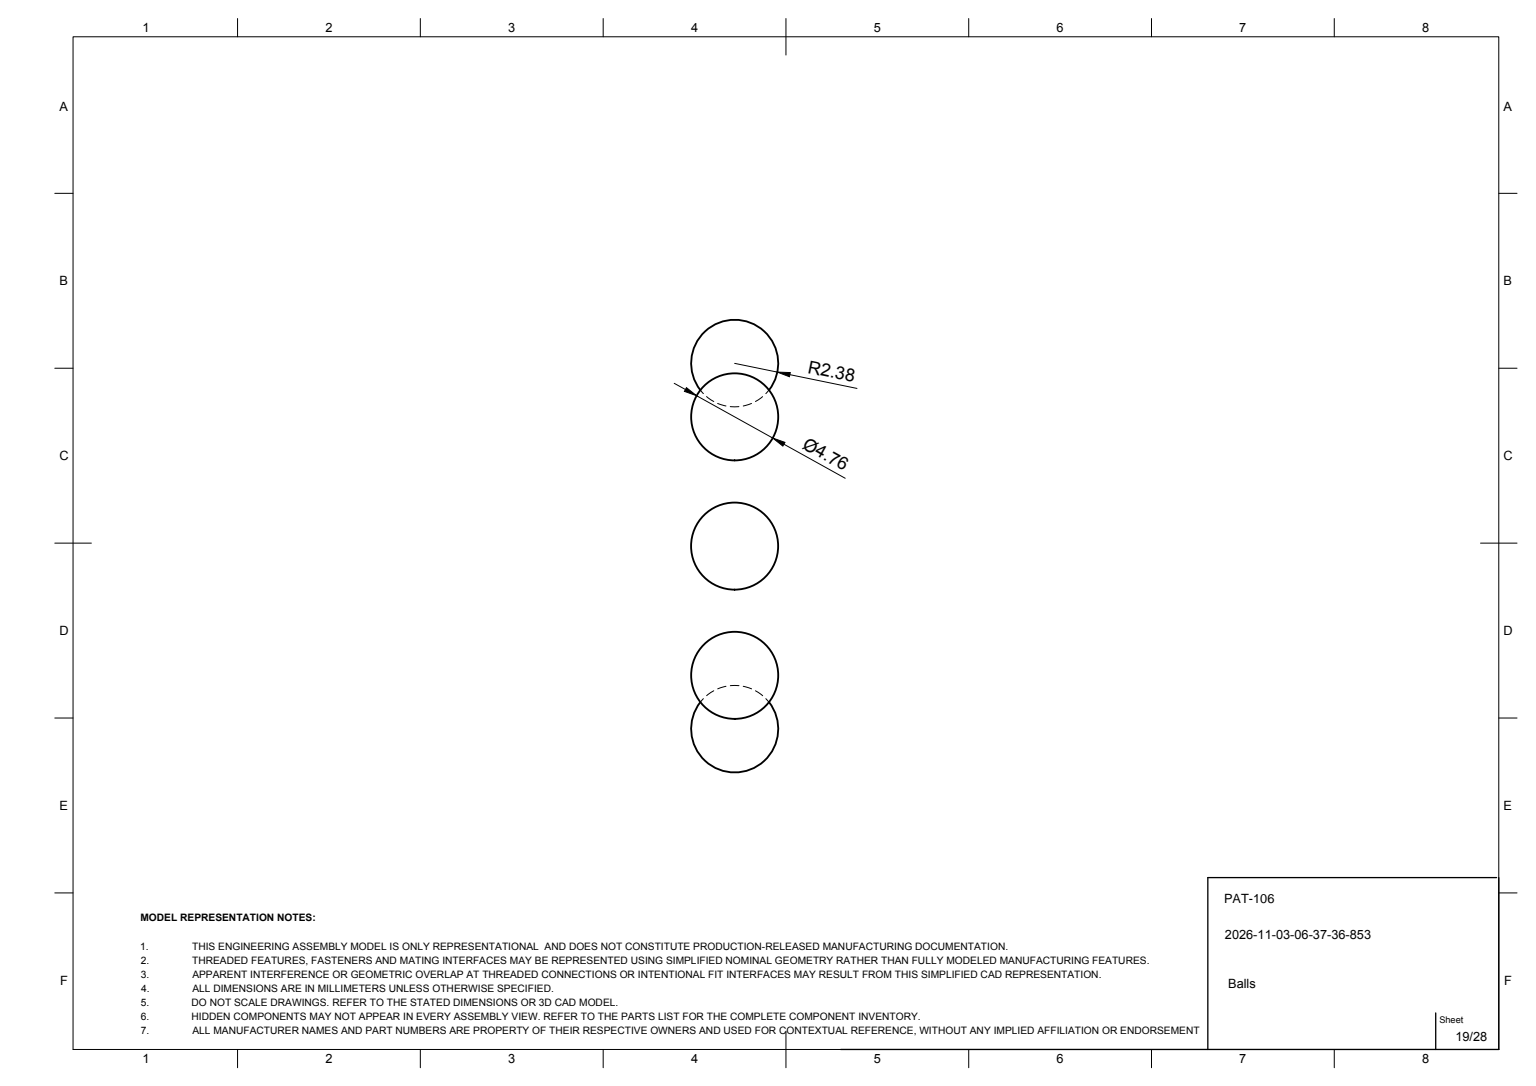
ISO-10303-21;
HEADER;
/* Generated by software containing ST-Developer
 * from STEP Tools, Inc. (www.steptools.com) 
 */

FILE_DESCRIPTION(
/* description */ ('Torsion-spring ratchet demonstrator'),
/* implementation_level */ '2;1');

FILE_NAME(
/* name */ 'Balls.step',
/* time_stamp */ '2026-10-29T17:29:17-07:00',
/* author */ (''),
/* organization */ (''),
/* preprocessor_version */ 'ST-DEVELOPER v20.2',
/* originating_system */ 'Autodesk Translation Framework v15.17.0.0',
/* authorisation */ '');

FILE_SCHEMA (('AUTOMOTIVE_DESIGN { 1 0 10303 214 3 1 1 }'));
ENDSEC;

DATA;
#10=MECHANICAL_DESIGN_GEOMETRIC_PRESENTATION_REPRESENTATION('',(#294,#295,#296,#297,#298,#299,#300,#301),#11258);
#170=SPHERICAL_SURFACE('',#5722,0.23815);
#171=SPHERICAL_SURFACE('',#5724,0.23815);
#172=SPHERICAL_SURFACE('',#5726,0.23815);
#173=SPHERICAL_SURFACE('',#5728,0.23815);
#174=SPHERICAL_SURFACE('',#5730,0.23815);
#175=SPHERICAL_SURFACE('',#5732,0.23815);
#176=SPHERICAL_SURFACE('',#5734,0.23815);
#177=SPHERICAL_SURFACE('',#5736,0.23815);
#246=SHAPE_REPRESENTATION_RELATIONSHIP('SRR','None',#11373,#270);
#270=ADVANCED_BREP_SHAPE_REPRESENTATION('',(#326,#327,#328,#329,#330,#331,
#332,#333),#11243);
#294=STYLED_ITEM('',(#11584),#326);
#295=STYLED_ITEM('',(#11584),#327);
#296=STYLED_ITEM('',(#11584),#328);
#297=STYLED_ITEM('',(#11584),#329);
#298=STYLED_ITEM('',(#11584),#330);
#299=STYLED_ITEM('',(#11584),#331);
#300=STYLED_ITEM('',(#11584),#332);
#301=STYLED_ITEM('',(#11584),#333);
#326=MANIFOLD_SOLID_BREP('Body1',#5165);
#327=MANIFOLD_SOLID_BREP('Body2',#5166);
#328=MANIFOLD_SOLID_BREP('Body3',#5167);
#329=MANIFOLD_SOLID_BREP('Body4',#5168);
#330=MANIFOLD_SOLID_BREP('Body5',#5169);
#331=MANIFOLD_SOLID_BREP('Body6',#5170);
#332=MANIFOLD_SOLID_BREP('Body7',#5171);
#333=MANIFOLD_SOLID_BREP('Body8',#5172);
#743=FACE_OUTER_BOUND('',#1116,.T.);
#744=FACE_OUTER_BOUND('',#1117,.T.);
#745=FACE_OUTER_BOUND('',#1118,.T.);
#746=FACE_OUTER_BOUND('',#1119,.T.);
#747=FACE_OUTER_BOUND('',#1120,.T.);
#748=FACE_OUTER_BOUND('',#1121,.T.);
#749=FACE_OUTER_BOUND('',#1122,.T.);
#750=FACE_OUTER_BOUND('',#1123,.T.);
#1116=EDGE_LOOP('',(#3926,#3927));
#1117=EDGE_LOOP('',(#3928,#3929));
#1118=EDGE_LOOP('',(#3930,#3931));
#1119=EDGE_LOOP('',(#3932,#3933));
#1120=EDGE_LOOP('',(#3934,#3935));
#1121=EDGE_LOOP('',(#3936,#3937));
#1122=EDGE_LOOP('',(#3938,#3939));
#1123=EDGE_LOOP('',(#3940,#3941));
#2225=CIRCLE('',#5723,0.23815);
#2226=CIRCLE('',#5725,0.23815);
#2227=CIRCLE('',#5727,0.23815);
#2228=CIRCLE('',#5729,0.23815);
#2229=CIRCLE('',#5731,0.23815);
#2230=CIRCLE('',#5733,0.23815);
#2231=CIRCLE('',#5735,0.23815);
#2232=CIRCLE('',#5737,0.23815);
#2495=VERTEX_POINT('',#8281);
#2496=VERTEX_POINT('',#8282);
#2497=VERTEX_POINT('',#8285);
#2498=VERTEX_POINT('',#8286);
#2499=VERTEX_POINT('',#8289);
#2500=VERTEX_POINT('',#8290);
#2501=VERTEX_POINT('',#8293);
#2502=VERTEX_POINT('',#8294);
#2503=VERTEX_POINT('',#8297);
#2504=VERTEX_POINT('',#8298);
#2505=VERTEX_POINT('',#8301);
#2506=VERTEX_POINT('',#8302);
#2507=VERTEX_POINT('',#8305);
#2508=VERTEX_POINT('',#8306);
#2509=VERTEX_POINT('',#8309);
#2510=VERTEX_POINT('',#8310);
#3023=EDGE_CURVE('',#2495,#2496,#2225,.T.);
#3024=EDGE_CURVE('',#2497,#2498,#2226,.T.);
#3025=EDGE_CURVE('',#2499,#2500,#2227,.T.);
#3026=EDGE_CURVE('',#2501,#2502,#2228,.T.);
#3027=EDGE_CURVE('',#2503,#2504,#2229,.T.);
#3028=EDGE_CURVE('',#2505,#2506,#2230,.T.);
#3029=EDGE_CURVE('',#2507,#2508,#2231,.T.);
#3030=EDGE_CURVE('',#2509,#2510,#2232,.T.);
#3926=ORIENTED_EDGE('',*,*,#3023,.T.);
#3927=ORIENTED_EDGE('',*,*,#3023,.F.);
#3928=ORIENTED_EDGE('',*,*,#3024,.T.);
#3929=ORIENTED_EDGE('',*,*,#3024,.F.);
#3930=ORIENTED_EDGE('',*,*,#3025,.T.);
#3931=ORIENTED_EDGE('',*,*,#3025,.F.);
#3932=ORIENTED_EDGE('',*,*,#3026,.T.);
#3933=ORIENTED_EDGE('',*,*,#3026,.F.);
#3934=ORIENTED_EDGE('',*,*,#3027,.T.);
#3935=ORIENTED_EDGE('',*,*,#3027,.F.);
#3936=ORIENTED_EDGE('',*,*,#3028,.T.);
#3937=ORIENTED_EDGE('',*,*,#3028,.F.);
#3938=ORIENTED_EDGE('',*,*,#3029,.T.);
#3939=ORIENTED_EDGE('',*,*,#3029,.F.);
#3940=ORIENTED_EDGE('',*,*,#3030,.T.);
#3941=ORIENTED_EDGE('',*,*,#3030,.F.);
#4969=ADVANCED_FACE('',(#743),#170,.T.);
#4970=ADVANCED_FACE('',(#744),#171,.T.);
#4971=ADVANCED_FACE('',(#745),#172,.T.);
#4972=ADVANCED_FACE('',(#746),#173,.T.);
#4973=ADVANCED_FACE('',(#747),#174,.T.);
#4974=ADVANCED_FACE('',(#748),#175,.T.);
#4975=ADVANCED_FACE('',(#749),#176,.T.);
#4976=ADVANCED_FACE('',(#750),#177,.T.);
#5165=CLOSED_SHELL('',(#4969));
#5166=CLOSED_SHELL('',(#4970));
#5167=CLOSED_SHELL('',(#4971));
#5168=CLOSED_SHELL('',(#4972));
#5169=CLOSED_SHELL('',(#4973));
#5170=CLOSED_SHELL('',(#4974));
#5171=CLOSED_SHELL('',(#4975));
#5172=CLOSED_SHELL('',(#4976));
#5721=AXIS2_PLACEMENT_3D('',#8279,#6706,#6707);
#5722=AXIS2_PLACEMENT_3D('',#8280,#6708,#6709);
#5723=AXIS2_PLACEMENT_3D('',#8283,#6710,#6711);
#5724=AXIS2_PLACEMENT_3D('',#8284,#6712,#6713);
#5725=AXIS2_PLACEMENT_3D('',#8287,#6714,#6715);
#5726=AXIS2_PLACEMENT_3D('',#8288,#6716,#6717);
#5727=AXIS2_PLACEMENT_3D('',#8291,#6718,#6719);
#5728=AXIS2_PLACEMENT_3D('',#8292,#6720,#6721);
#5729=AXIS2_PLACEMENT_3D('',#8295,#6722,#6723);
#5730=AXIS2_PLACEMENT_3D('',#8296,#6724,#6725);
#5731=AXIS2_PLACEMENT_3D('',#8299,#6726,#6727);
#5732=AXIS2_PLACEMENT_3D('',#8300,#6728,#6729);
#5733=AXIS2_PLACEMENT_3D('',#8303,#6730,#6731);
#5734=AXIS2_PLACEMENT_3D('',#8304,#6732,#6733);
#5735=AXIS2_PLACEMENT_3D('',#8307,#6734,#6735);
#5736=AXIS2_PLACEMENT_3D('',#8308,#6736,#6737);
#5737=AXIS2_PLACEMENT_3D('',#8311,#6738,#6739);
#6706=DIRECTION('axis',(0.,0.,1.));
#6707=DIRECTION('refdir',(1.,0.,0.));
#6708=DIRECTION('center_axis',(0.,0.,1.));
#6709=DIRECTION('ref_axis',(1.,0.,0.));
#6710=DIRECTION('center_axis',(1.22464679914735E-16,-1.,0.));
#6711=DIRECTION('ref_axis',(-1.,-1.22464679914735E-16,0.));
#6712=DIRECTION('center_axis',(0.707106781186548,0.,0.707106781186548));
#6713=DIRECTION('ref_axis',(0.707106781186548,0.,-0.707106781186548));
#6714=DIRECTION('center_axis',(8.65956056235494E-17,-1.,-8.65956056235493E-17));
#6715=DIRECTION('ref_axis',(-0.707106781186547,-1.22464679914735E-16,0.707106781186547));
#6716=DIRECTION('center_axis',(1.,0.,0.));
#6717=DIRECTION('ref_axis',(6.12323399573676E-17,0.,-1.));
#6718=DIRECTION('center_axis',(7.49879891330929E-33,-1.,-1.22464679914735E-16));
#6719=DIRECTION('ref_axis',(-6.12323399573676E-17,-1.22464679914735E-16,
1.));
#6720=DIRECTION('center_axis',(0.707106781186548,0.,-0.707106781186548));
#6721=DIRECTION('ref_axis',(-0.707106781186548,0.,-0.707106781186548));
#6722=DIRECTION('center_axis',(-8.65956056235493E-17,-1.,-8.65956056235494E-17));
#6723=DIRECTION('ref_axis',(0.707106781186547,-1.22464679914735E-16,0.707106781186547));
#6724=DIRECTION('center_axis',(0.,0.,-1.));
#6725=DIRECTION('ref_axis',(-1.,0.,-1.22464679914735E-16));
#6726=DIRECTION('center_axis',(-1.22464679914735E-16,-1.,-1.49975978266186E-32));
#6727=DIRECTION('ref_axis',(1.,-1.22464679914735E-16,1.22464679914735E-16));
#6728=DIRECTION('center_axis',(-0.707106781186547,0.,-0.707106781186548));
#6729=DIRECTION('ref_axis',(-0.707106781186548,0.,0.707106781186547));
#6730=DIRECTION('center_axis',(-8.65956056235493E-17,-1.,8.65956056235493E-17));
#6731=DIRECTION('ref_axis',(0.707106781186548,-1.22464679914735E-16,-0.707106781186547));
#6732=DIRECTION('center_axis',(-1.,0.,0.));
#6733=DIRECTION('ref_axis',(-1.83697019872103E-16,0.,1.));
#6734=DIRECTION('center_axis',(-2.24963967399279E-32,-1.,1.22464679914735E-16));
#6735=DIRECTION('ref_axis',(1.83697019872103E-16,-1.22464679914735E-16,
-1.));
#6736=DIRECTION('center_axis',(-0.707106781186548,0.,0.707106781186548));
#6737=DIRECTION('ref_axis',(0.707106781186547,0.,0.707106781186548));
#6738=DIRECTION('center_axis',(8.65956056235493E-17,-1.,8.65956056235493E-17));
#6739=DIRECTION('ref_axis',(-0.707106781186547,-1.22464679914735E-16,-0.707106781186548));
#8279=CARTESIAN_POINT('',(0.,0.,0.));
#8280=CARTESIAN_POINT('Origin',(1.,0.,0.));
#8281=CARTESIAN_POINT('',(1.,-1.78583896120461E-33,0.23815));
#8282=CARTESIAN_POINT('',(1.,-1.78583896120461E-33,-0.23815));
#8283=CARTESIAN_POINT('Origin',(1.,0.,0.));
#8284=CARTESIAN_POINT('Origin',(0.707106781186548,0.,-0.707106781186547));
#8285=CARTESIAN_POINT('',(0.875504261126124,-1.78583896120461E-33,-0.538709301246971));
#8286=CARTESIAN_POINT('',(0.538709301246971,-1.78583896120461E-33,-0.875504261126124));
#8287=CARTESIAN_POINT('Origin',(0.707106781186548,0.,-0.707106781186547));
#8288=CARTESIAN_POINT('Origin',(6.12323399573677E-17,0.,-1.));
#8289=CARTESIAN_POINT('',(0.23815,-1.78583896120461E-33,-1.));
#8290=CARTESIAN_POINT('',(-0.23815,-1.78583896120461E-33,-1.));
#8291=CARTESIAN_POINT('Origin',(6.12323399573677E-17,0.,-1.));
#8292=CARTESIAN_POINT('Origin',(-0.707106781186547,0.,-0.707106781186548));
#8293=CARTESIAN_POINT('',(-0.538709301246971,-1.78583896120461E-33,-0.875504261126124));
#8294=CARTESIAN_POINT('',(-0.875504261126124,-1.78583896120461E-33,-0.538709301246971));
#8295=CARTESIAN_POINT('Origin',(-0.707106781186547,0.,-0.707106781186548));
#8296=CARTESIAN_POINT('Origin',(-1.,0.,-1.22464679914735E-16));
#8297=CARTESIAN_POINT('',(-1.,-1.78583896120461E-33,-0.23815));
#8298=CARTESIAN_POINT('',(-1.,-1.78583896120461E-33,0.23815));
#8299=CARTESIAN_POINT('Origin',(-1.,0.,-1.22464679914735E-16));
#8300=CARTESIAN_POINT('Origin',(-0.707106781186548,0.,0.707106781186547));
#8301=CARTESIAN_POINT('',(-0.875504261126124,-7.94881478324376E-33,0.538709301246971));
#8302=CARTESIAN_POINT('',(-0.538709301246971,4.37713686083455E-33,0.875504261126124));
#8303=CARTESIAN_POINT('Origin',(-0.707106781186548,0.,0.707106781186547));
#8304=CARTESIAN_POINT('Origin',(-1.83697019872103E-16,0.,1.));
#8305=CARTESIAN_POINT('',(-0.23815,-1.78583896120461E-33,1.));
#8306=CARTESIAN_POINT('',(0.23815,-1.78583896120461E-33,1.));
#8307=CARTESIAN_POINT('Origin',(-1.83697019872103E-16,0.,1.));
#8308=CARTESIAN_POINT('Origin',(0.707106781186547,0.,0.707106781186548));
#8309=CARTESIAN_POINT('',(0.538709301246971,-4.86732687222419E-33,0.875504261126124));
#8310=CARTESIAN_POINT('',(0.875504261126124,1.29564894981497E-33,0.538709301246971));
#8311=CARTESIAN_POINT('Origin',(0.707106781186547,0.,0.707106781186548));
#11213=UNCERTAINTY_MEASURE_WITH_UNIT(LENGTH_MEASURE(0.001),#11259,
'DISTANCE_ACCURACY_VALUE',
'Maximum model space distance between geometric entities at asserted c
onnectivities');
#11228=UNCERTAINTY_MEASURE_WITH_UNIT(LENGTH_MEASURE(0.001),#11259,
'DISTANCE_ACCURACY_VALUE',
'Maximum model space distance between geometric entities at asserted c
onnectivities');
#11243=(
GEOMETRIC_REPRESENTATION_CONTEXT(3)
GLOBAL_UNCERTAINTY_ASSIGNED_CONTEXT((#11213))
GLOBAL_UNIT_ASSIGNED_CONTEXT((#11259,#11261,#11262))
REPRESENTATION_CONTEXT('','3D')
);
#11258=(
GEOMETRIC_REPRESENTATION_CONTEXT(3)
GLOBAL_UNCERTAINTY_ASSIGNED_CONTEXT((#11228))
GLOBAL_UNIT_ASSIGNED_CONTEXT((#11259,#11261,#11262))
REPRESENTATION_CONTEXT('','3D')
);
#11259=(
LENGTH_UNIT()
NAMED_UNIT(*)
SI_UNIT(.CENTI.,.METRE.)
);
#11261=(
NAMED_UNIT(*)
PLANE_ANGLE_UNIT()
SI_UNIT($,.RADIAN.)
);
#11262=(
NAMED_UNIT(*)
SI_UNIT($,.STERADIAN.)
SOLID_ANGLE_UNIT()
);
#11277=SHAPE_DEFINITION_REPRESENTATION(#11306,#11373);
#11306=PRODUCT_DEFINITION_SHAPE('',$,#11403);
#11373=SHAPE_REPRESENTATION('',(#5721),#11243);
#11388=PRODUCT_DEFINITION_CONTEXT('part definition',#11477,'design');
#11403=PRODUCT_DEFINITION('Balls','Balls',#11432,#11388);
#11432=PRODUCT_DEFINITION_FORMATION('',$,#11493);
#11477=APPLICATION_CONTEXT(
'Core Data for Automotive Mechanical Design Process');
#11478=PRODUCT_CONTEXT('part definition',#11477,'mechanical');
#11493=PRODUCT('Balls','Balls','Balls',(#11478));
#11578=COLOUR_RGB('Grey',0.48,0.52,0.57);
#11579=FILL_AREA_STYLE_COLOUR('',#11578);
#11580=FILL_AREA_STYLE('',(#11579));
#11581=SURFACE_STYLE_FILL_AREA(#11580);
#11582=SURFACE_SIDE_STYLE('',(#11581));
#11583=SURFACE_STYLE_USAGE(.BOTH.,#11582);
#11584=PRESENTATION_STYLE_ASSIGNMENT((#11583));
ENDSEC;
END-ISO-10303-21;
